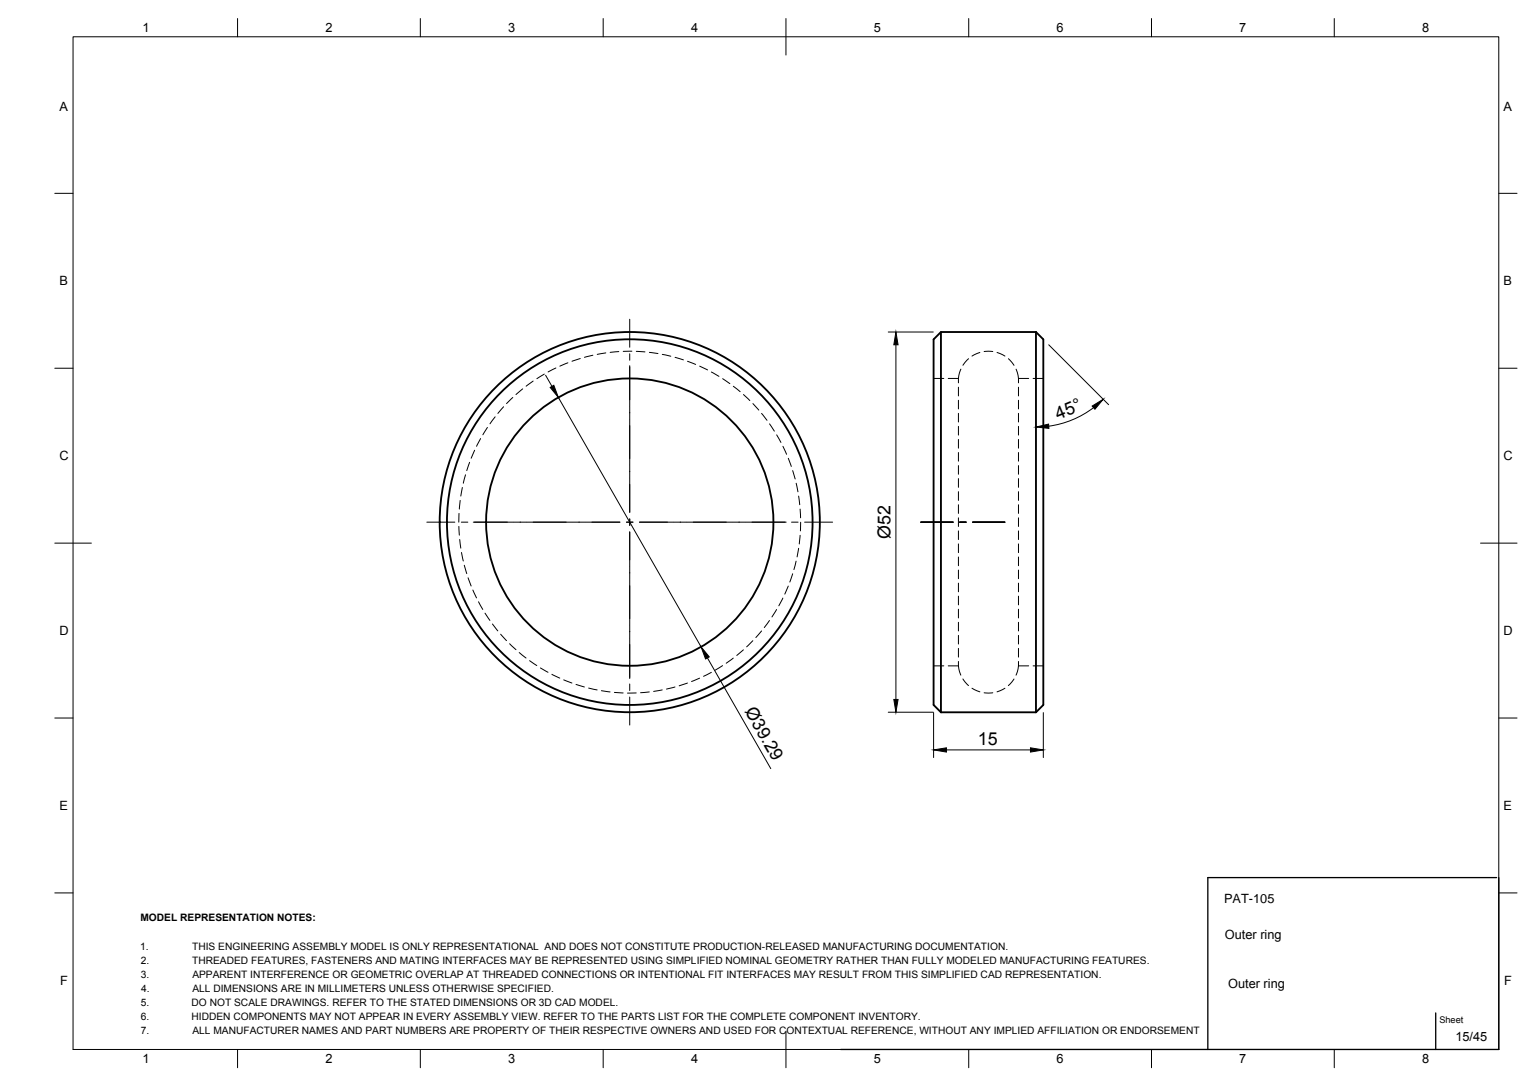
ISO-10303-21;
HEADER;
/* Generated by software containing ST-Developer
 * from STEP Tools, Inc. (www.steptools.com) 
 */

FILE_DESCRIPTION(
/* description */ ('Torque wrench calibration arm'),
/* implementation_level */ '2;1');

FILE_NAME(
/* name */ 'Outer ring.step',
/* time_stamp */ '2026-10-28T03:24:52-07:00',
/* author */ (''),
/* organization */ (''),
/* preprocessor_version */ 'ST-DEVELOPER v20.2',
/* originating_system */ 'Autodesk Translation Framework v15.17.0.0',
/* authorisation */ '');

FILE_SCHEMA (('AUTOMOTIVE_DESIGN { 1 0 10303 214 3 1 1 }'));
ENDSEC;

DATA;
#10=MECHANICAL_DESIGN_GEOMETRIC_PRESENTATION_REPRESENTATION('',(#434),#12783);
#329=CONICAL_SURFACE('',#7190,2.55,0.785398163397449);
#330=CONICAL_SURFACE('',#7194,2.55,0.785398163397449);
#349=TOROIDAL_SURFACE('',#7179,1.925,0.412776);
#360=SHAPE_REPRESENTATION_RELATIONSHIP('SRR','None',#12942,#397);
#397=ADVANCED_BREP_SHAPE_REPRESENTATION('',(#488),#12751);
#434=STYLED_ITEM('',(#13212),#488);
#488=MANIFOLD_SOLID_BREP('Body1',#6503);
#585=FACE_BOUND('',#1435,.T.);
#586=FACE_BOUND('',#1440,.T.);
#712=PLANE('',#7187);
#713=PLANE('',#7196);
#983=FACE_OUTER_BOUND('',#1432,.T.);
#984=FACE_OUTER_BOUND('',#1433,.T.);
#985=FACE_OUTER_BOUND('',#1434,.T.);
#986=FACE_OUTER_BOUND('',#1436,.T.);
#987=FACE_OUTER_BOUND('',#1437,.T.);
#988=FACE_OUTER_BOUND('',#1438,.T.);
#989=FACE_OUTER_BOUND('',#1439,.T.);
#990=FACE_OUTER_BOUND('',#1441,.T.);
#1432=EDGE_LOOP('',(#4827,#4828,#4829,#4830,#4831,#4832));
#1433=EDGE_LOOP('',(#4833,#4834,#4835,#4836,#4837));
#1434=EDGE_LOOP('',(#4838));
#1435=EDGE_LOOP('',(#4839));
#1436=EDGE_LOOP('',(#4840,#4841,#4842,#4843));
#1437=EDGE_LOOP('',(#4844,#4845,#4846,#4847));
#1438=EDGE_LOOP('',(#4848,#4849,#4850,#4851));
#1439=EDGE_LOOP('',(#4852));
#1440=EDGE_LOOP('',(#4853));
#1441=EDGE_LOOP('',(#4854,#4855,#4856,#4857,#4858));
#1925=LINE('',#10454,#2340);
#1926=LINE('',#10463,#2341);
#1927=LINE('',#10467,#2342);
#1928=LINE('',#10471,#2343);
#1929=LINE('',#10474,#2344);
#2340=VECTOR('',#8403,1.96469);
#2341=VECTOR('',#8414,2.55);
#2342=VECTOR('',#8419,2.6);
#2343=VECTOR('',#8424,2.55);
#2344=VECTOR('',#8429,1.96469);
#2715=CIRCLE('',#7180,1.96469);
#2716=CIRCLE('',#7181,1.96469);
#2717=CIRCLE('',#7182,0.412776);
#2718=CIRCLE('',#7183,1.96469);
#2719=CIRCLE('',#7184,1.96469);
#2720=CIRCLE('',#7186,1.96469);
#2721=CIRCLE('',#7188,2.5);
#2722=CIRCLE('',#7189,1.96469);
#2723=CIRCLE('',#7191,2.6);
#2724=CIRCLE('',#7193,2.6);
#2725=CIRCLE('',#7195,2.5);
#3129=VERTEX_POINT('',#10442);
#3130=VERTEX_POINT('',#10443);
#3131=VERTEX_POINT('',#10446);
#3132=VERTEX_POINT('',#10448);
#3133=VERTEX_POINT('',#10452);
#3134=VERTEX_POINT('',#10456);
#3135=VERTEX_POINT('',#10458);
#3136=VERTEX_POINT('',#10461);
#3137=VERTEX_POINT('',#10465);
#3138=VERTEX_POINT('',#10469);
#3771=EDGE_CURVE('',#3129,#3130,#2715,.T.);
#3772=EDGE_CURVE('',#3130,#3129,#2716,.T.);
#3773=EDGE_CURVE('',#3130,#3131,#2717,.T.);
#3774=EDGE_CURVE('',#3132,#3131,#2718,.T.);
#3775=EDGE_CURVE('',#3131,#3132,#2719,.T.);
#3776=EDGE_CURVE('',#3133,#3133,#2720,.T.);
#3777=EDGE_CURVE('',#3133,#3132,#1925,.T.);
#3778=EDGE_CURVE('',#3134,#3134,#2721,.T.);
#3779=EDGE_CURVE('',#3135,#3135,#2722,.T.);
#3780=EDGE_CURVE('',#3136,#3136,#2723,.T.);
#3781=EDGE_CURVE('',#3136,#3134,#1926,.T.);
#3782=EDGE_CURVE('',#3137,#3137,#2724,.T.);
#3783=EDGE_CURVE('',#3137,#3136,#1927,.T.);
#3784=EDGE_CURVE('',#3138,#3138,#2725,.T.);
#3785=EDGE_CURVE('',#3138,#3137,#1928,.T.);
#3786=EDGE_CURVE('',#3129,#3135,#1929,.T.);
#4827=ORIENTED_EDGE('',*,*,#3771,.F.);
#4828=ORIENTED_EDGE('',*,*,#3772,.F.);
#4829=ORIENTED_EDGE('',*,*,#3773,.T.);
#4830=ORIENTED_EDGE('',*,*,#3774,.F.);
#4831=ORIENTED_EDGE('',*,*,#3775,.F.);
#4832=ORIENTED_EDGE('',*,*,#3773,.F.);
#4833=ORIENTED_EDGE('',*,*,#3776,.T.);
#4834=ORIENTED_EDGE('',*,*,#3777,.T.);
#4835=ORIENTED_EDGE('',*,*,#3774,.T.);
#4836=ORIENTED_EDGE('',*,*,#3775,.T.);
#4837=ORIENTED_EDGE('',*,*,#3777,.F.);
#4838=ORIENTED_EDGE('',*,*,#3778,.F.);
#4839=ORIENTED_EDGE('',*,*,#3779,.T.);
#4840=ORIENTED_EDGE('',*,*,#3780,.F.);
#4841=ORIENTED_EDGE('',*,*,#3781,.T.);
#4842=ORIENTED_EDGE('',*,*,#3778,.T.);
#4843=ORIENTED_EDGE('',*,*,#3781,.F.);
#4844=ORIENTED_EDGE('',*,*,#3782,.F.);
#4845=ORIENTED_EDGE('',*,*,#3783,.T.);
#4846=ORIENTED_EDGE('',*,*,#3780,.T.);
#4847=ORIENTED_EDGE('',*,*,#3783,.F.);
#4848=ORIENTED_EDGE('',*,*,#3784,.F.);
#4849=ORIENTED_EDGE('',*,*,#3785,.T.);
#4850=ORIENTED_EDGE('',*,*,#3782,.T.);
#4851=ORIENTED_EDGE('',*,*,#3785,.F.);
#4852=ORIENTED_EDGE('',*,*,#3784,.T.);
#4853=ORIENTED_EDGE('',*,*,#3776,.F.);
#4854=ORIENTED_EDGE('',*,*,#3771,.T.);
#4855=ORIENTED_EDGE('',*,*,#3772,.T.);
#4856=ORIENTED_EDGE('',*,*,#3786,.T.);
#4857=ORIENTED_EDGE('',*,*,#3779,.F.);
#4858=ORIENTED_EDGE('',*,*,#3786,.F.);
#6032=CYLINDRICAL_SURFACE('',#7185,1.96469);
#6033=CYLINDRICAL_SURFACE('',#7192,2.6);
#6034=CYLINDRICAL_SURFACE('',#7197,1.96469);
#6208=ADVANCED_FACE('',(#983),#349,.F.);
#6209=ADVANCED_FACE('',(#984),#6032,.F.);
#6210=ADVANCED_FACE('',(#985,#585),#712,.T.);
#6211=ADVANCED_FACE('',(#986),#329,.T.);
#6212=ADVANCED_FACE('',(#987),#6033,.T.);
#6213=ADVANCED_FACE('',(#988),#330,.T.);
#6214=ADVANCED_FACE('',(#989,#586),#713,.T.);
#6215=ADVANCED_FACE('',(#990),#6034,.F.);
#6503=CLOSED_SHELL('',(#6208,#6209,#6210,#6211,#6212,#6213,#6214,#6215));
#7178=AXIS2_PLACEMENT_3D('',#10440,#8385,#8386);
#7179=AXIS2_PLACEMENT_3D('',#10441,#8387,#8388);
#7180=AXIS2_PLACEMENT_3D('',#10444,#8389,#8390);
#7181=AXIS2_PLACEMENT_3D('',#10445,#8391,#8392);
#7182=AXIS2_PLACEMENT_3D('',#10447,#8393,#8394);
#7183=AXIS2_PLACEMENT_3D('',#10449,#8395,#8396);
#7184=AXIS2_PLACEMENT_3D('',#10450,#8397,#8398);
#7185=AXIS2_PLACEMENT_3D('',#10451,#8399,#8400);
#7186=AXIS2_PLACEMENT_3D('',#10453,#8401,#8402);
#7187=AXIS2_PLACEMENT_3D('',#10455,#8404,#8405);
#7188=AXIS2_PLACEMENT_3D('',#10457,#8406,#8407);
#7189=AXIS2_PLACEMENT_3D('',#10459,#8408,#8409);
#7190=AXIS2_PLACEMENT_3D('',#10460,#8410,#8411);
#7191=AXIS2_PLACEMENT_3D('',#10462,#8412,#8413);
#7192=AXIS2_PLACEMENT_3D('',#10464,#8415,#8416);
#7193=AXIS2_PLACEMENT_3D('',#10466,#8417,#8418);
#7194=AXIS2_PLACEMENT_3D('',#10468,#8420,#8421);
#7195=AXIS2_PLACEMENT_3D('',#10470,#8422,#8423);
#7196=AXIS2_PLACEMENT_3D('',#10472,#8425,#8426);
#7197=AXIS2_PLACEMENT_3D('',#10473,#8427,#8428);
#8385=DIRECTION('axis',(0.,0.,1.));
#8386=DIRECTION('refdir',(1.,0.,0.));
#8387=DIRECTION('center_axis',(0.,-1.,0.));
#8388=DIRECTION('ref_axis',(0.,0.,-1.));
#8389=DIRECTION('center_axis',(0.,-1.,0.));
#8390=DIRECTION('ref_axis',(1.,0.,0.));
#8391=DIRECTION('center_axis',(0.,-1.,0.));
#8392=DIRECTION('ref_axis',(1.,0.,0.));
#8393=DIRECTION('center_axis',(1.,0.,1.22464679914735E-16));
#8394=DIRECTION('ref_axis',(-1.22464679914735E-16,0.,1.));
#8395=DIRECTION('center_axis',(0.,1.,0.));
#8396=DIRECTION('ref_axis',(1.,0.,0.));
#8397=DIRECTION('center_axis',(0.,1.,0.));
#8398=DIRECTION('ref_axis',(1.,0.,0.));
#8399=DIRECTION('center_axis',(0.,-1.,0.));
#8400=DIRECTION('ref_axis',(1.,0.,0.));
#8401=DIRECTION('center_axis',(0.,-1.,0.));
#8402=DIRECTION('ref_axis',(1.,0.,0.));
#8403=DIRECTION('',(0.,1.,0.));
#8404=DIRECTION('center_axis',(0.,1.,0.));
#8405=DIRECTION('ref_axis',(0.,0.,1.));
#8406=DIRECTION('center_axis',(0.,-1.,0.));
#8407=DIRECTION('ref_axis',(1.,0.,0.));
#8408=DIRECTION('center_axis',(0.,-1.,0.));
#8409=DIRECTION('ref_axis',(1.,0.,0.));
#8410=DIRECTION('center_axis',(0.,-1.,0.));
#8411=DIRECTION('ref_axis',(1.,0.,0.));
#8412=DIRECTION('center_axis',(0.,-1.,0.));
#8413=DIRECTION('ref_axis',(1.,0.,0.));
#8414=DIRECTION('',(0.707106781186548,0.707106781186547,8.65956056235494E-17));
#8415=DIRECTION('center_axis',(0.,-1.,0.));
#8416=DIRECTION('ref_axis',(1.,0.,0.));
#8417=DIRECTION('center_axis',(0.,-1.,0.));
#8418=DIRECTION('ref_axis',(1.,0.,0.));
#8419=DIRECTION('',(0.,1.,0.));
#8420=DIRECTION('center_axis',(0.,1.,0.));
#8421=DIRECTION('ref_axis',(1.,0.,0.));
#8422=DIRECTION('center_axis',(0.,-1.,0.));
#8423=DIRECTION('ref_axis',(1.,0.,0.));
#8424=DIRECTION('',(-0.707106781186548,0.707106781186547,-8.65956056235494E-17));
#8425=DIRECTION('center_axis',(0.,-1.,0.));
#8426=DIRECTION('ref_axis',(0.,0.,-1.));
#8427=DIRECTION('center_axis',(0.,-1.,0.));
#8428=DIRECTION('ref_axis',(1.,0.,0.));
#8429=DIRECTION('',(0.,1.,0.));
#10440=CARTESIAN_POINT('',(0.,0.,0.));
#10441=CARTESIAN_POINT('Origin',(0.,0.,0.));
#10442=CARTESIAN_POINT('',(-1.96469,0.410863395882378,-2.40605131981681E-16));
#10443=CARTESIAN_POINT('',(-2.40605131981681E-16,0.410863395882378,1.96469));
#10444=CARTESIAN_POINT('Origin',(0.,0.410863395882378,0.));
#10445=CARTESIAN_POINT('Origin',(0.,0.410863395882378,0.));
#10446=CARTESIAN_POINT('',(-2.40605131981681E-16,-0.410863395882378,1.96469));
#10447=CARTESIAN_POINT('Origin',(-2.35744508835865E-16,0.,1.925));
#10448=CARTESIAN_POINT('',(-1.96469,-0.410863395882378,2.40605131981681E-16));
#10449=CARTESIAN_POINT('Origin',(0.,-0.410863395882378,0.));
#10450=CARTESIAN_POINT('Origin',(0.,-0.410863395882378,0.));
#10451=CARTESIAN_POINT('Origin',(0.,0.,0.));
#10452=CARTESIAN_POINT('',(-1.96469,-0.75,-2.40605131981681E-16));
#10453=CARTESIAN_POINT('Origin',(0.,-0.75,0.));
#10454=CARTESIAN_POINT('',(-1.96469,0.,-2.40605131981681E-16));
#10455=CARTESIAN_POINT('Origin',(2.5,0.75,0.));
#10456=CARTESIAN_POINT('',(-2.5,0.75,-3.06161699786838E-16));
#10457=CARTESIAN_POINT('Origin',(0.,0.75,0.));
#10458=CARTESIAN_POINT('',(-1.96469,0.75,-2.40605131981681E-16));
#10459=CARTESIAN_POINT('Origin',(0.,0.75,0.));
#10460=CARTESIAN_POINT('Origin',(0.,0.7,0.));
#10461=CARTESIAN_POINT('',(-2.6,0.65,-3.18408167778312E-16));
#10462=CARTESIAN_POINT('Origin',(0.,0.65,0.));
#10463=CARTESIAN_POINT('',(-2.55,0.7,-3.12284933782575E-16));
#10464=CARTESIAN_POINT('Origin',(0.,0.,0.));
#10465=CARTESIAN_POINT('',(-2.6,-0.65,-3.18408167778312E-16));
#10466=CARTESIAN_POINT('Origin',(0.,-0.65,0.));
#10467=CARTESIAN_POINT('',(-2.6,0.,-3.18408167778312E-16));
#10468=CARTESIAN_POINT('Origin',(0.,-0.7,0.));
#10469=CARTESIAN_POINT('',(-2.5,-0.75,-3.06161699786838E-16));
#10470=CARTESIAN_POINT('Origin',(0.,-0.75,0.));
#10471=CARTESIAN_POINT('',(-2.55,-0.7,-3.12284933782575E-16));
#10472=CARTESIAN_POINT('Origin',(1.96469,-0.75,0.));
#10473=CARTESIAN_POINT('Origin',(0.,0.,0.));
#10474=CARTESIAN_POINT('',(-1.96469,0.,-2.40605131981681E-16));
#12707=UNCERTAINTY_MEASURE_WITH_UNIT(LENGTH_MEASURE(0.001),#12784,
'DISTANCE_ACCURACY_VALUE',
'Maximum model space distance between geometric entities at asserted c
onnectivities');
#12739=UNCERTAINTY_MEASURE_WITH_UNIT(LENGTH_MEASURE(0.001),#12784,
'DISTANCE_ACCURACY_VALUE',
'Maximum model space distance between geometric entities at asserted c
onnectivities');
#12751=(
GEOMETRIC_REPRESENTATION_CONTEXT(3)
GLOBAL_UNCERTAINTY_ASSIGNED_CONTEXT((#12707))
GLOBAL_UNIT_ASSIGNED_CONTEXT((#12784,#12786,#12787))
REPRESENTATION_CONTEXT('','3D')
);
#12783=(
GEOMETRIC_REPRESENTATION_CONTEXT(3)
GLOBAL_UNCERTAINTY_ASSIGNED_CONTEXT((#12739))
GLOBAL_UNIT_ASSIGNED_CONTEXT((#12784,#12786,#12787))
REPRESENTATION_CONTEXT('','3D')
);
#12784=(
LENGTH_UNIT()
NAMED_UNIT(*)
SI_UNIT(.CENTI.,.METRE.)
);
#12786=(
NAMED_UNIT(*)
PLANE_ANGLE_UNIT()
SI_UNIT($,.RADIAN.)
);
#12787=(
NAMED_UNIT(*)
SI_UNIT($,.STERADIAN.)
SOLID_ANGLE_UNIT()
);
#12799=SHAPE_DEFINITION_REPRESENTATION(#12842,#12942);
#12842=PRODUCT_DEFINITION_SHAPE('',$,#12986);
#12942=SHAPE_REPRESENTATION('',(#7178),#12751);
#12974=PRODUCT_DEFINITION_CONTEXT('part definition',#13105,'design');
#12986=PRODUCT_DEFINITION('Outer ring','Outer ring',#13029,#12974);
#13029=PRODUCT_DEFINITION_FORMATION('',$,#13118);
#13105=APPLICATION_CONTEXT(
'Core Data for Automotive Mechanical Design Process');
#13106=PRODUCT_CONTEXT('part definition',#13105,'mechanical');
#13118=PRODUCT('Outer ring','Outer ring','Outer ring',(#13106));
#13206=COLOUR_RGB('Grey',0.48,0.52,0.57);
#13207=FILL_AREA_STYLE_COLOUR('',#13206);
#13208=FILL_AREA_STYLE('',(#13207));
#13209=SURFACE_STYLE_FILL_AREA(#13208);
#13210=SURFACE_SIDE_STYLE('',(#13209));
#13211=SURFACE_STYLE_USAGE(.BOTH.,#13210);
#13212=PRESENTATION_STYLE_ASSIGNMENT((#13211));
ENDSEC;
END-ISO-10303-21;
